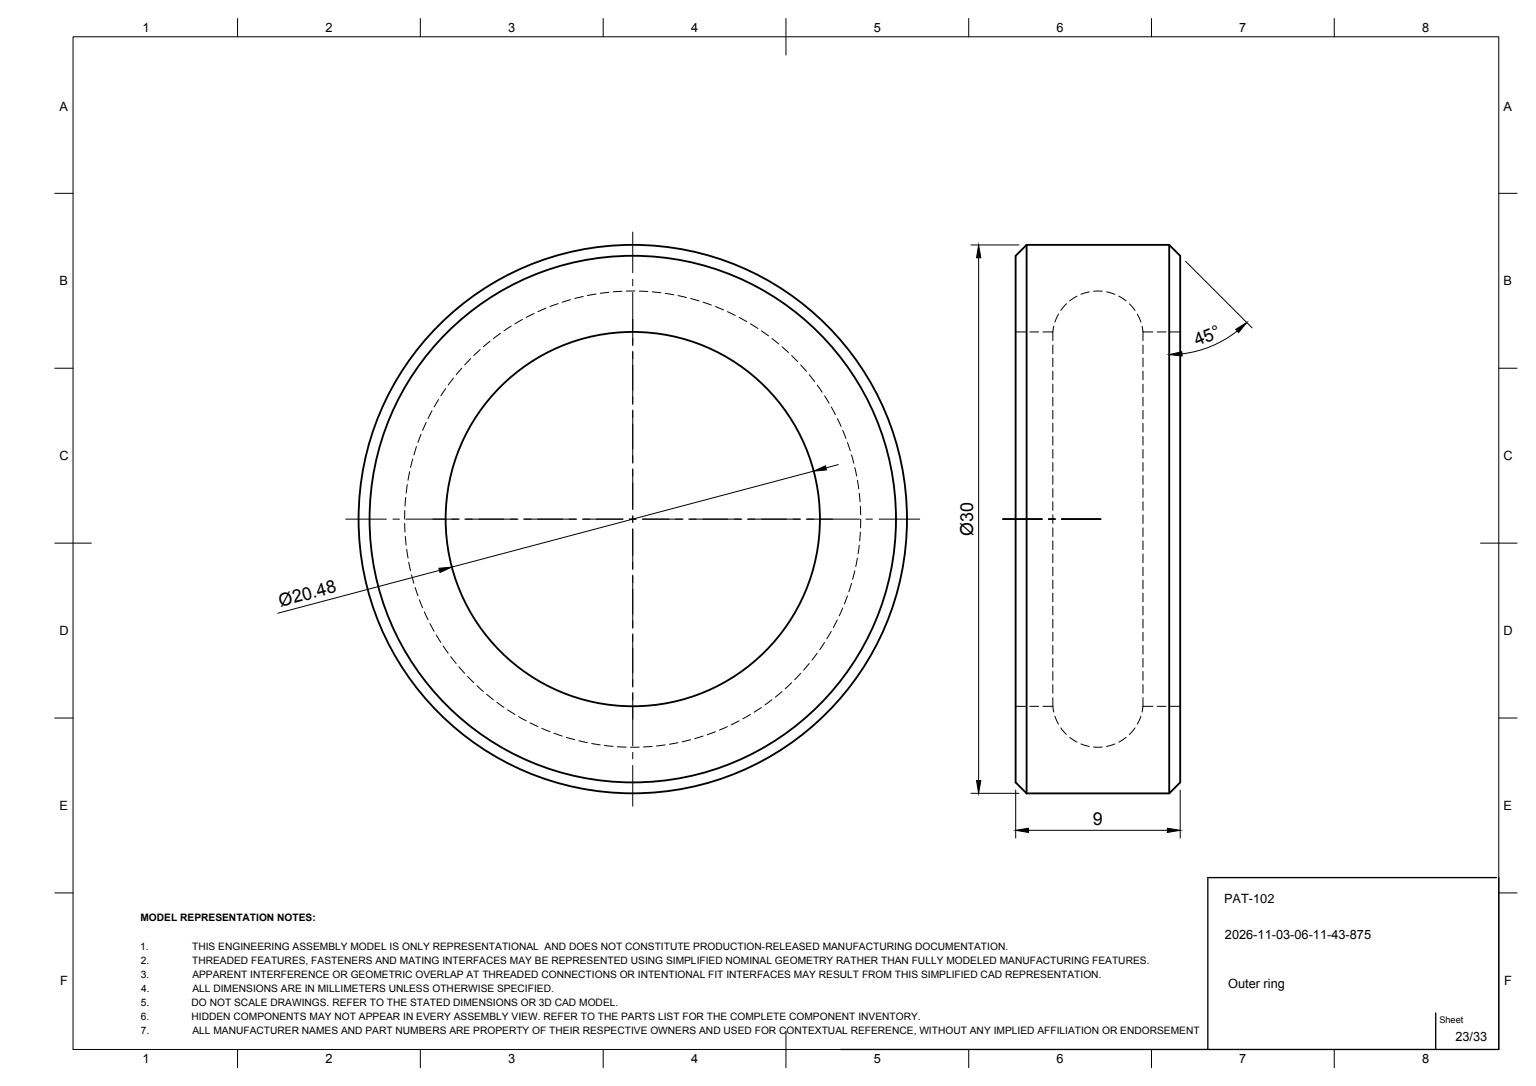
ISO-10303-21;
HEADER;
/* Generated by software containing ST-Developer
 * from STEP Tools, Inc. (www.steptools.com) 
 */

FILE_DESCRIPTION(
/* description */ ('Swing-away clamp arm'),
/* implementation_level */ '2;1');

FILE_NAME(
/* name */ 'Outer ring.step',
/* time_stamp */ '2026-10-28T03:26:03-07:00',
/* author */ (''),
/* organization */ (''),
/* preprocessor_version */ 'ST-DEVELOPER v20.2',
/* originating_system */ 'Autodesk Translation Framework v15.17.0.0',
/* authorisation */ '');

FILE_SCHEMA (('AUTOMOTIVE_DESIGN { 1 0 10303 214 3 1 1 }'));
ENDSEC;

DATA;
#10=MECHANICAL_DESIGN_GEOMETRIC_PRESENTATION_REPRESENTATION('',(#308),#10627);
#28=TOROIDAL_SURFACE('',#5601,1.,0.247676);
#206=CONICAL_SURFACE('',#5612,1.47,0.785398163397449);
#207=CONICAL_SURFACE('',#5616,1.47,0.785398163397449);
#256=SHAPE_REPRESENTATION_RELATIONSHIP('SRR','None',#10756,#282);
#282=ADVANCED_BREP_SHAPE_REPRESENTATION('',(#341),#10615);
#308=STYLED_ITEM('',(#10965),#341);
#341=MANIFOLD_SOLID_BREP('Body1',#4915);
#434=FACE_BOUND('',#1217,.T.);
#435=FACE_BOUND('',#1222,.T.);
#580=PLANE('',#5609);
#581=PLANE('',#5618);
#831=FACE_OUTER_BOUND('',#1214,.T.);
#832=FACE_OUTER_BOUND('',#1215,.T.);
#833=FACE_OUTER_BOUND('',#1216,.T.);
#834=FACE_OUTER_BOUND('',#1218,.T.);
#835=FACE_OUTER_BOUND('',#1219,.T.);
#836=FACE_OUTER_BOUND('',#1220,.T.);
#837=FACE_OUTER_BOUND('',#1221,.T.);
#838=FACE_OUTER_BOUND('',#1223,.T.);
#1214=EDGE_LOOP('',(#4073,#4074,#4075,#4076,#4077,#4078));
#1215=EDGE_LOOP('',(#4079,#4080,#4081,#4082,#4083));
#1216=EDGE_LOOP('',(#4084));
#1217=EDGE_LOOP('',(#4085));
#1218=EDGE_LOOP('',(#4086,#4087,#4088,#4089));
#1219=EDGE_LOOP('',(#4090,#4091,#4092,#4093));
#1220=EDGE_LOOP('',(#4094,#4095,#4096,#4097));
#1221=EDGE_LOOP('',(#4098));
#1222=EDGE_LOOP('',(#4099));
#1223=EDGE_LOOP('',(#4100,#4101,#4102,#4103,#4104));
#1591=LINE('',#9721,#1913);
#1592=LINE('',#9730,#1914);
#1593=LINE('',#9734,#1915);
#1594=LINE('',#9738,#1916);
#1595=LINE('',#9741,#1917);
#1913=VECTOR('',#6882,1.023815);
#1914=VECTOR('',#6893,1.47);
#1915=VECTOR('',#6898,1.5);
#1916=VECTOR('',#6903,1.47);
#1917=VECTOR('',#6908,1.023815);
#2150=CIRCLE('',#5602,1.023815);
#2151=CIRCLE('',#5603,1.023815);
#2152=CIRCLE('',#5604,0.247676);
#2153=CIRCLE('',#5605,1.023815);
#2154=CIRCLE('',#5606,1.023815);
#2155=CIRCLE('',#5608,1.023815);
#2156=CIRCLE('',#5610,1.44);
#2157=CIRCLE('',#5611,1.023815);
#2158=CIRCLE('',#5613,1.5);
#2159=CIRCLE('',#5615,1.5);
#2160=CIRCLE('',#5617,1.44);
#2524=VERTEX_POINT('',#9709);
#2525=VERTEX_POINT('',#9710);
#2526=VERTEX_POINT('',#9713);
#2527=VERTEX_POINT('',#9715);
#2528=VERTEX_POINT('',#9719);
#2529=VERTEX_POINT('',#9723);
#2530=VERTEX_POINT('',#9725);
#2531=VERTEX_POINT('',#9728);
#2532=VERTEX_POINT('',#9732);
#2533=VERTEX_POINT('',#9736);
#3069=EDGE_CURVE('',#2524,#2525,#2150,.T.);
#3070=EDGE_CURVE('',#2525,#2524,#2151,.T.);
#3071=EDGE_CURVE('',#2525,#2526,#2152,.T.);
#3072=EDGE_CURVE('',#2527,#2526,#2153,.T.);
#3073=EDGE_CURVE('',#2526,#2527,#2154,.T.);
#3074=EDGE_CURVE('',#2528,#2528,#2155,.T.);
#3075=EDGE_CURVE('',#2528,#2527,#1591,.T.);
#3076=EDGE_CURVE('',#2529,#2529,#2156,.T.);
#3077=EDGE_CURVE('',#2530,#2530,#2157,.T.);
#3078=EDGE_CURVE('',#2531,#2531,#2158,.T.);
#3079=EDGE_CURVE('',#2531,#2529,#1592,.T.);
#3080=EDGE_CURVE('',#2532,#2532,#2159,.T.);
#3081=EDGE_CURVE('',#2532,#2531,#1593,.T.);
#3082=EDGE_CURVE('',#2533,#2533,#2160,.T.);
#3083=EDGE_CURVE('',#2533,#2532,#1594,.T.);
#3084=EDGE_CURVE('',#2524,#2530,#1595,.T.);
#4073=ORIENTED_EDGE('',*,*,#3069,.F.);
#4074=ORIENTED_EDGE('',*,*,#3070,.F.);
#4075=ORIENTED_EDGE('',*,*,#3071,.T.);
#4076=ORIENTED_EDGE('',*,*,#3072,.F.);
#4077=ORIENTED_EDGE('',*,*,#3073,.F.);
#4078=ORIENTED_EDGE('',*,*,#3071,.F.);
#4079=ORIENTED_EDGE('',*,*,#3074,.T.);
#4080=ORIENTED_EDGE('',*,*,#3075,.T.);
#4081=ORIENTED_EDGE('',*,*,#3072,.T.);
#4082=ORIENTED_EDGE('',*,*,#3073,.T.);
#4083=ORIENTED_EDGE('',*,*,#3075,.F.);
#4084=ORIENTED_EDGE('',*,*,#3076,.F.);
#4085=ORIENTED_EDGE('',*,*,#3077,.T.);
#4086=ORIENTED_EDGE('',*,*,#3078,.F.);
#4087=ORIENTED_EDGE('',*,*,#3079,.T.);
#4088=ORIENTED_EDGE('',*,*,#3076,.T.);
#4089=ORIENTED_EDGE('',*,*,#3079,.F.);
#4090=ORIENTED_EDGE('',*,*,#3080,.F.);
#4091=ORIENTED_EDGE('',*,*,#3081,.T.);
#4092=ORIENTED_EDGE('',*,*,#3078,.T.);
#4093=ORIENTED_EDGE('',*,*,#3081,.F.);
#4094=ORIENTED_EDGE('',*,*,#3082,.F.);
#4095=ORIENTED_EDGE('',*,*,#3083,.T.);
#4096=ORIENTED_EDGE('',*,*,#3080,.T.);
#4097=ORIENTED_EDGE('',*,*,#3083,.F.);
#4098=ORIENTED_EDGE('',*,*,#3082,.T.);
#4099=ORIENTED_EDGE('',*,*,#3074,.F.);
#4100=ORIENTED_EDGE('',*,*,#3069,.T.);
#4101=ORIENTED_EDGE('',*,*,#3070,.T.);
#4102=ORIENTED_EDGE('',*,*,#3084,.T.);
#4103=ORIENTED_EDGE('',*,*,#3077,.F.);
#4104=ORIENTED_EDGE('',*,*,#3084,.F.);
#4562=CYLINDRICAL_SURFACE('',#5607,1.023815);
#4563=CYLINDRICAL_SURFACE('',#5614,1.5);
#4564=CYLINDRICAL_SURFACE('',#5619,1.023815);
#4786=ADVANCED_FACE('',(#831),#28,.F.);
#4787=ADVANCED_FACE('',(#832),#4562,.F.);
#4788=ADVANCED_FACE('',(#833,#434),#580,.T.);
#4789=ADVANCED_FACE('',(#834),#206,.T.);
#4790=ADVANCED_FACE('',(#835),#4563,.T.);
#4791=ADVANCED_FACE('',(#836),#207,.T.);
#4792=ADVANCED_FACE('',(#837,#435),#581,.T.);
#4793=ADVANCED_FACE('',(#838),#4564,.F.);
#4915=CLOSED_SHELL('',(#4786,#4787,#4788,#4789,#4790,#4791,#4792,#4793));
#5600=AXIS2_PLACEMENT_3D('',#9707,#6864,#6865);
#5601=AXIS2_PLACEMENT_3D('',#9708,#6866,#6867);
#5602=AXIS2_PLACEMENT_3D('',#9711,#6868,#6869);
#5603=AXIS2_PLACEMENT_3D('',#9712,#6870,#6871);
#5604=AXIS2_PLACEMENT_3D('',#9714,#6872,#6873);
#5605=AXIS2_PLACEMENT_3D('',#9716,#6874,#6875);
#5606=AXIS2_PLACEMENT_3D('',#9717,#6876,#6877);
#5607=AXIS2_PLACEMENT_3D('',#9718,#6878,#6879);
#5608=AXIS2_PLACEMENT_3D('',#9720,#6880,#6881);
#5609=AXIS2_PLACEMENT_3D('',#9722,#6883,#6884);
#5610=AXIS2_PLACEMENT_3D('',#9724,#6885,#6886);
#5611=AXIS2_PLACEMENT_3D('',#9726,#6887,#6888);
#5612=AXIS2_PLACEMENT_3D('',#9727,#6889,#6890);
#5613=AXIS2_PLACEMENT_3D('',#9729,#6891,#6892);
#5614=AXIS2_PLACEMENT_3D('',#9731,#6894,#6895);
#5615=AXIS2_PLACEMENT_3D('',#9733,#6896,#6897);
#5616=AXIS2_PLACEMENT_3D('',#9735,#6899,#6900);
#5617=AXIS2_PLACEMENT_3D('',#9737,#6901,#6902);
#5618=AXIS2_PLACEMENT_3D('',#9739,#6904,#6905);
#5619=AXIS2_PLACEMENT_3D('',#9740,#6906,#6907);
#6864=DIRECTION('axis',(0.,0.,1.));
#6865=DIRECTION('refdir',(1.,0.,0.));
#6866=DIRECTION('center_axis',(0.,-1.,0.));
#6867=DIRECTION('ref_axis',(0.,0.,-1.));
#6868=DIRECTION('center_axis',(0.,-1.,0.));
#6869=DIRECTION('ref_axis',(1.,0.,0.));
#6870=DIRECTION('center_axis',(0.,-1.,0.));
#6871=DIRECTION('ref_axis',(1.,0.,0.));
#6872=DIRECTION('center_axis',(1.,0.,1.22464679914735E-16));
#6873=DIRECTION('ref_axis',(-1.22464679914735E-16,0.,1.));
#6874=DIRECTION('center_axis',(0.,1.,0.));
#6875=DIRECTION('ref_axis',(1.,0.,0.));
#6876=DIRECTION('center_axis',(0.,1.,0.));
#6877=DIRECTION('ref_axis',(1.,0.,0.));
#6878=DIRECTION('center_axis',(0.,-1.,0.));
#6879=DIRECTION('ref_axis',(1.,0.,0.));
#6880=DIRECTION('center_axis',(0.,-1.,0.));
#6881=DIRECTION('ref_axis',(1.,0.,0.));
#6882=DIRECTION('',(0.,1.,0.));
#6883=DIRECTION('center_axis',(0.,1.,0.));
#6884=DIRECTION('ref_axis',(0.,0.,1.));
#6885=DIRECTION('center_axis',(0.,-1.,0.));
#6886=DIRECTION('ref_axis',(1.,0.,0.));
#6887=DIRECTION('center_axis',(0.,-1.,0.));
#6888=DIRECTION('ref_axis',(1.,0.,0.));
#6889=DIRECTION('center_axis',(0.,-1.,0.));
#6890=DIRECTION('ref_axis',(1.,0.,0.));
#6891=DIRECTION('center_axis',(0.,-1.,0.));
#6892=DIRECTION('ref_axis',(1.,0.,0.));
#6893=DIRECTION('',(0.707106781186548,0.707106781186547,8.65956056235494E-17));
#6894=DIRECTION('center_axis',(0.,-1.,0.));
#6895=DIRECTION('ref_axis',(1.,0.,0.));
#6896=DIRECTION('center_axis',(0.,-1.,0.));
#6897=DIRECTION('ref_axis',(1.,0.,0.));
#6898=DIRECTION('',(0.,1.,0.));
#6899=DIRECTION('center_axis',(0.,1.,0.));
#6900=DIRECTION('ref_axis',(1.,0.,0.));
#6901=DIRECTION('center_axis',(0.,-1.,0.));
#6902=DIRECTION('ref_axis',(1.,0.,0.));
#6903=DIRECTION('',(-0.707106781186548,0.707106781186547,-8.65956056235494E-17));
#6904=DIRECTION('center_axis',(0.,-1.,0.));
#6905=DIRECTION('ref_axis',(0.,0.,-1.));
#6906=DIRECTION('center_axis',(0.,-1.,0.));
#6907=DIRECTION('ref_axis',(1.,0.,0.));
#6908=DIRECTION('',(0.,1.,0.));
#9707=CARTESIAN_POINT('',(0.,0.,0.));
#9708=CARTESIAN_POINT('Origin',(0.,0.,0.));
#9709=CARTESIAN_POINT('',(-1.023815,0.246528389340863,-1.25381176266905E-16));
#9710=CARTESIAN_POINT('',(-1.25381176266905E-16,0.246528389340863,1.023815));
#9711=CARTESIAN_POINT('Origin',(0.,0.246528389340863,0.));
#9712=CARTESIAN_POINT('Origin',(0.,0.246528389340863,0.));
#9713=CARTESIAN_POINT('',(-1.25381176266905E-16,-0.246528389340863,1.023815));
#9714=CARTESIAN_POINT('Origin',(-1.22464679914735E-16,0.,1.));
#9715=CARTESIAN_POINT('',(-1.023815,-0.246528389340863,1.25381176266905E-16));
#9716=CARTESIAN_POINT('Origin',(0.,-0.246528389340863,0.));
#9717=CARTESIAN_POINT('Origin',(0.,-0.246528389340863,0.));
#9718=CARTESIAN_POINT('Origin',(0.,0.,0.));
#9719=CARTESIAN_POINT('',(-1.023815,-0.45,-1.25381176266905E-16));
#9720=CARTESIAN_POINT('Origin',(0.,-0.45,0.));
#9721=CARTESIAN_POINT('',(-1.023815,0.,-1.25381176266905E-16));
#9722=CARTESIAN_POINT('Origin',(1.44,0.45,0.));
#9723=CARTESIAN_POINT('',(-1.44,0.45,-1.76349139077219E-16));
#9724=CARTESIAN_POINT('Origin',(0.,0.45,0.));
#9725=CARTESIAN_POINT('',(-1.023815,0.45,-1.25381176266905E-16));
#9726=CARTESIAN_POINT('Origin',(0.,0.45,0.));
#9727=CARTESIAN_POINT('Origin',(0.,0.42,0.));
#9728=CARTESIAN_POINT('',(-1.5,0.39,-1.83697019872103E-16));
#9729=CARTESIAN_POINT('Origin',(0.,0.39,0.));
#9730=CARTESIAN_POINT('',(-1.47,0.42,-1.80023079474661E-16));
#9731=CARTESIAN_POINT('Origin',(0.,0.,0.));
#9732=CARTESIAN_POINT('',(-1.5,-0.39,-1.83697019872103E-16));
#9733=CARTESIAN_POINT('Origin',(0.,-0.39,0.));
#9734=CARTESIAN_POINT('',(-1.5,0.,-1.83697019872103E-16));
#9735=CARTESIAN_POINT('Origin',(0.,-0.42,0.));
#9736=CARTESIAN_POINT('',(-1.44,-0.45,-1.76349139077219E-16));
#9737=CARTESIAN_POINT('Origin',(0.,-0.45,0.));
#9738=CARTESIAN_POINT('',(-1.47,-0.42,-1.80023079474661E-16));
#9739=CARTESIAN_POINT('Origin',(1.023815,-0.45,0.));
#9740=CARTESIAN_POINT('Origin',(0.,0.,0.));
#9741=CARTESIAN_POINT('',(-1.023815,0.,-1.25381176266905E-16));
#10583=UNCERTAINTY_MEASURE_WITH_UNIT(LENGTH_MEASURE(0.001),#10628,
'DISTANCE_ACCURACY_VALUE',
'Maximum model space distance between geometric entities at asserted c
onnectivities');
#10595=UNCERTAINTY_MEASURE_WITH_UNIT(LENGTH_MEASURE(0.001),#10628,
'DISTANCE_ACCURACY_VALUE',
'Maximum model space distance between geometric entities at asserted c
onnectivities');
#10615=(
GEOMETRIC_REPRESENTATION_CONTEXT(3)
GLOBAL_UNCERTAINTY_ASSIGNED_CONTEXT((#10583))
GLOBAL_UNIT_ASSIGNED_CONTEXT((#10628,#10630,#10631))
REPRESENTATION_CONTEXT('','3D')
);
#10627=(
GEOMETRIC_REPRESENTATION_CONTEXT(3)
GLOBAL_UNCERTAINTY_ASSIGNED_CONTEXT((#10595))
GLOBAL_UNIT_ASSIGNED_CONTEXT((#10628,#10630,#10631))
REPRESENTATION_CONTEXT('','3D')
);
#10628=(
LENGTH_UNIT()
NAMED_UNIT(*)
SI_UNIT(.CENTI.,.METRE.)
);
#10630=(
NAMED_UNIT(*)
PLANE_ANGLE_UNIT()
SI_UNIT($,.RADIAN.)
);
#10631=(
NAMED_UNIT(*)
SI_UNIT($,.STERADIAN.)
SOLID_ANGLE_UNIT()
);
#10651=SHAPE_DEFINITION_REPRESENTATION(#10692,#10756);
#10692=PRODUCT_DEFINITION_SHAPE('',$,#10788);
#10756=SHAPE_REPRESENTATION('',(#5600),#10615);
#10768=PRODUCT_DEFINITION_CONTEXT('part definition',#10863,'design');
#10788=PRODUCT_DEFINITION('Outer ring','Outer ring',#10819,#10768);
#10819=PRODUCT_DEFINITION_FORMATION('',$,#10884);
#10863=APPLICATION_CONTEXT(
'Core Data for Automotive Mechanical Design Process');
#10864=PRODUCT_CONTEXT('part definition',#10863,'mechanical');
#10884=PRODUCT('Outer ring','Outer ring','Outer ring',(#10864));
#10959=COLOUR_RGB('Grey',0.48,0.52,0.57);
#10960=FILL_AREA_STYLE_COLOUR('',#10959);
#10961=FILL_AREA_STYLE('',(#10960));
#10962=SURFACE_STYLE_FILL_AREA(#10961);
#10963=SURFACE_SIDE_STYLE('',(#10962));
#10964=SURFACE_STYLE_USAGE(.BOTH.,#10963);
#10965=PRESENTATION_STYLE_ASSIGNMENT((#10964));
ENDSEC;
END-ISO-10303-21;
